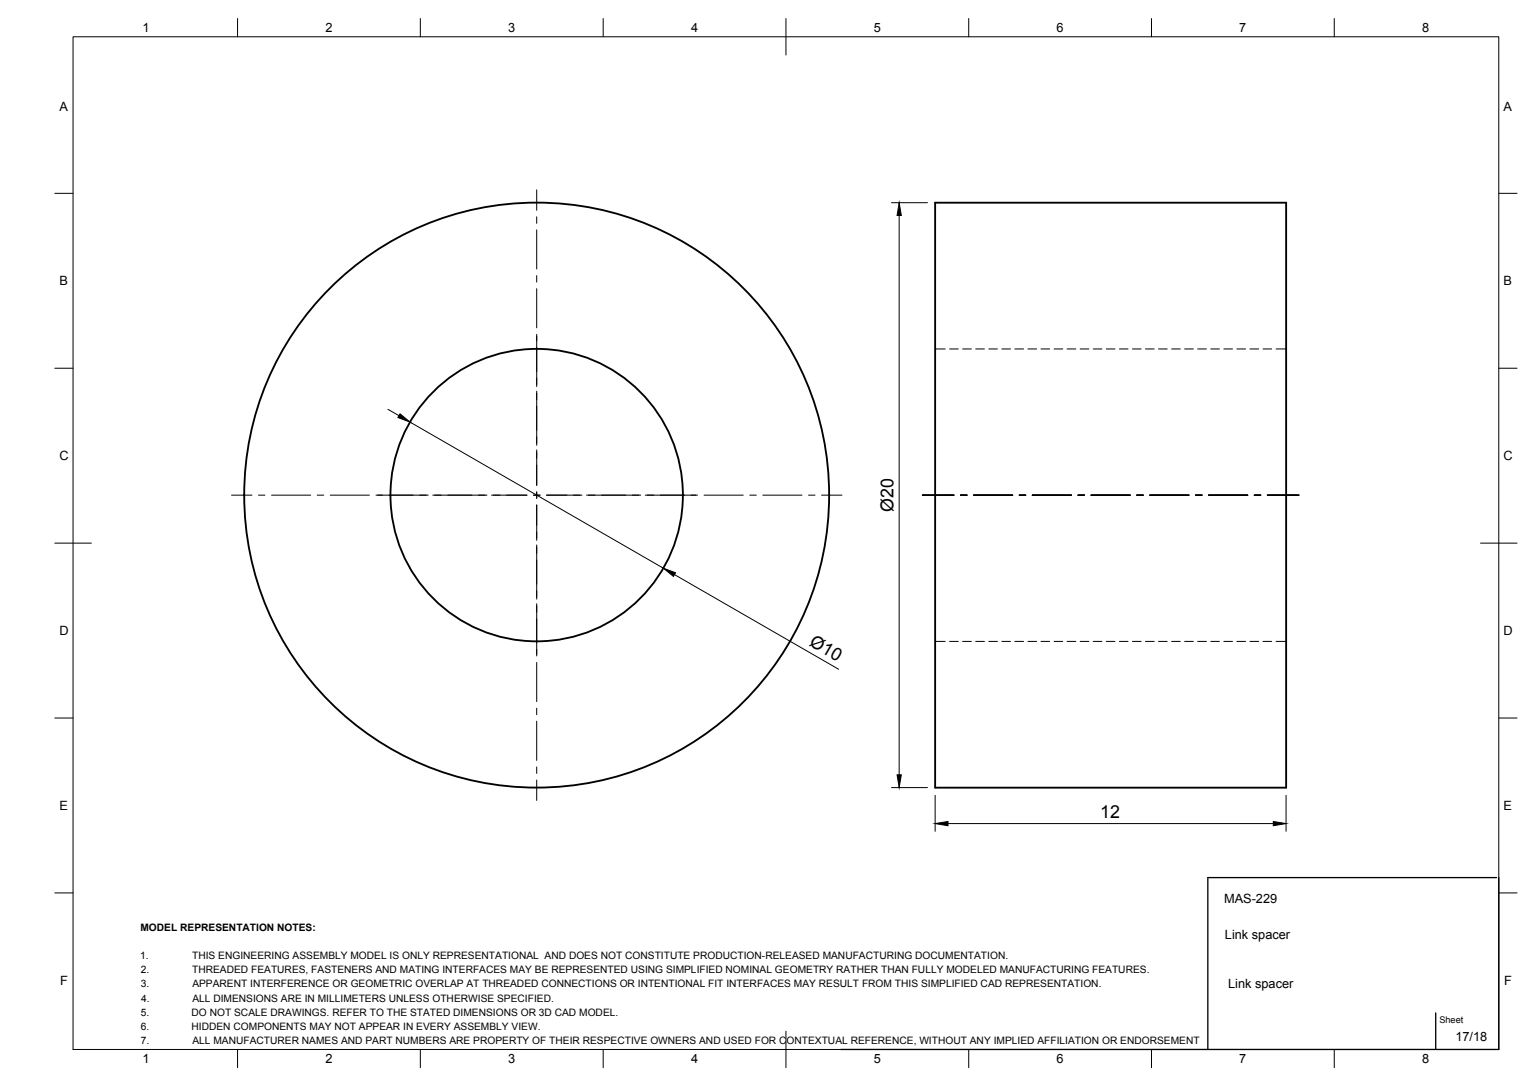
ISO-10303-21;
HEADER;
/* Generated by software containing ST-Developer
 * from STEP Tools, Inc. (www.steptools.com) 
 */

FILE_DESCRIPTION(
/* description */ ('Independently dimensioned six-bar single-leg walking-linkage demonstr
ator. Whole-mm20 crank,60 upper rocker,80/120 ternary coupler,120 lowe
r rocker,140 knee pitch and260 toe reach; ground pivots0/0,60/0,40/60.
 Seven native revolutes close both loops. Four reused native library f
amilies, fully retained shared pins and layered real spacer stacks, bo
nded rubber toe. Benchtop reference mechanism; no complete vehicle, lo
ad, gait stability, adhesive, weld, fit or life rating.'),
/* implementation_level */ '2;1');

FILE_NAME(
/* name */ 'Link spacer.step',
/* time_stamp */ '2026-11-09T20:33:14-08:00',
/* author */ (''),
/* organization */ (''),
/* preprocessor_version */ 'ST-DEVELOPER v20.2',
/* originating_system */ 'Autodesk Translation Framework v15.17.0.0',
/* authorisation */ '');

FILE_SCHEMA (('AUTOMOTIVE_DESIGN { 1 0 10303 214 3 1 1 }'));
ENDSEC;

DATA;
#10=MECHANICAL_DESIGN_GEOMETRIC_PRESENTATION_REPRESENTATION('',(#272),#4048);
#236=SHAPE_REPRESENTATION_RELATIONSHIP('SRR','None',#4160,#254);
#254=ADVANCED_BREP_SHAPE_REPRESENTATION('',(#290),#4047);
#272=STYLED_ITEM('',(#4253),#290);
#290=MANIFOLD_SOLID_BREP('Body1',#2161);
#346=FACE_BOUND('',#721,.T.);
#347=FACE_BOUND('',#723,.T.);
#413=PLANE('',#2618);
#414=PLANE('',#2619);
#537=FACE_OUTER_BOUND('',#718,.T.);
#538=FACE_OUTER_BOUND('',#719,.T.);
#539=FACE_OUTER_BOUND('',#720,.T.);
#540=FACE_OUTER_BOUND('',#722,.T.);
#718=EDGE_LOOP('',(#1951,#1952,#1953,#1954));
#719=EDGE_LOOP('',(#1955,#1956,#1957,#1958));
#720=EDGE_LOOP('',(#1959));
#721=EDGE_LOOP('',(#1960));
#722=EDGE_LOOP('',(#1961));
#723=EDGE_LOOP('',(#1962));
#847=LINE('',#3948,#972);
#848=LINE('',#3954,#973);
#972=VECTOR('',#3300,5.);
#973=VECTOR('',#3307,10.);
#1084=CIRCLE('',#2613,5.);
#1085=CIRCLE('',#2614,5.);
#1086=CIRCLE('',#2616,10.);
#1087=CIRCLE('',#2617,10.);
#1242=VERTEX_POINT('',#3945);
#1243=VERTEX_POINT('',#3947);
#1244=VERTEX_POINT('',#3951);
#1245=VERTEX_POINT('',#3953);
#1479=EDGE_CURVE('',#1242,#1242,#1084,.T.);
#1480=EDGE_CURVE('',#1242,#1243,#847,.T.);
#1481=EDGE_CURVE('',#1243,#1243,#1085,.T.);
#1482=EDGE_CURVE('',#1244,#1244,#1086,.T.);
#1483=EDGE_CURVE('',#1244,#1245,#848,.T.);
#1484=EDGE_CURVE('',#1245,#1245,#1087,.T.);
#1951=ORIENTED_EDGE('',*,*,#1479,.F.);
#1952=ORIENTED_EDGE('',*,*,#1480,.T.);
#1953=ORIENTED_EDGE('',*,*,#1481,.T.);
#1954=ORIENTED_EDGE('',*,*,#1480,.F.);
#1955=ORIENTED_EDGE('',*,*,#1482,.F.);
#1956=ORIENTED_EDGE('',*,*,#1483,.T.);
#1957=ORIENTED_EDGE('',*,*,#1484,.T.);
#1958=ORIENTED_EDGE('',*,*,#1483,.F.);
#1959=ORIENTED_EDGE('',*,*,#1482,.T.);
#1960=ORIENTED_EDGE('',*,*,#1479,.T.);
#1961=ORIENTED_EDGE('',*,*,#1484,.F.);
#1962=ORIENTED_EDGE('',*,*,#1481,.F.);
#2016=CYLINDRICAL_SURFACE('',#2612,5.);
#2017=CYLINDRICAL_SURFACE('',#2615,10.);
#2140=ADVANCED_FACE('',(#537),#2016,.F.);
#2141=ADVANCED_FACE('',(#538),#2017,.T.);
#2142=ADVANCED_FACE('',(#539,#346),#413,.T.);
#2143=ADVANCED_FACE('',(#540,#347),#414,.F.);
#2161=CLOSED_SHELL('',(#2140,#2141,#2142,#2143));
#2611=AXIS2_PLACEMENT_3D('',#3943,#3294,#3295);
#2612=AXIS2_PLACEMENT_3D('',#3944,#3296,#3297);
#2613=AXIS2_PLACEMENT_3D('',#3946,#3298,#3299);
#2614=AXIS2_PLACEMENT_3D('',#3949,#3301,#3302);
#2615=AXIS2_PLACEMENT_3D('',#3950,#3303,#3304);
#2616=AXIS2_PLACEMENT_3D('',#3952,#3305,#3306);
#2617=AXIS2_PLACEMENT_3D('',#3955,#3308,#3309);
#2618=AXIS2_PLACEMENT_3D('',#3956,#3310,#3311);
#2619=AXIS2_PLACEMENT_3D('',#3957,#3312,#3313);
#3294=DIRECTION('axis',(0.,0.,1.));
#3295=DIRECTION('refdir',(1.,0.,0.));
#3296=DIRECTION('center_axis',(0.,0.,1.));
#3297=DIRECTION('ref_axis',(1.,0.,0.));
#3298=DIRECTION('center_axis',(0.,0.,-1.));
#3299=DIRECTION('ref_axis',(1.,0.,0.));
#3300=DIRECTION('',(0.,0.,-1.));
#3301=DIRECTION('center_axis',(0.,0.,-1.));
#3302=DIRECTION('ref_axis',(1.,0.,0.));
#3303=DIRECTION('center_axis',(0.,0.,1.));
#3304=DIRECTION('ref_axis',(1.,0.,0.));
#3305=DIRECTION('center_axis',(0.,0.,1.));
#3306=DIRECTION('ref_axis',(1.,0.,0.));
#3307=DIRECTION('',(0.,0.,-1.));
#3308=DIRECTION('center_axis',(0.,0.,1.));
#3309=DIRECTION('ref_axis',(1.,0.,0.));
#3310=DIRECTION('center_axis',(0.,0.,1.));
#3311=DIRECTION('ref_axis',(1.,0.,0.));
#3312=DIRECTION('center_axis',(0.,0.,1.));
#3313=DIRECTION('ref_axis',(1.,0.,0.));
#3943=CARTESIAN_POINT('',(0.,0.,0.));
#3944=CARTESIAN_POINT('Origin',(0.,0.,0.));
#3945=CARTESIAN_POINT('',(-5.,-6.12323399573677E-16,12.));
#3946=CARTESIAN_POINT('Origin',(0.,0.,12.));
#3947=CARTESIAN_POINT('',(-5.,-6.12323399573677E-16,0.));
#3948=CARTESIAN_POINT('',(-5.,-6.12323399573677E-16,0.));
#3949=CARTESIAN_POINT('Origin',(0.,0.,0.));
#3950=CARTESIAN_POINT('Origin',(0.,0.,0.));
#3951=CARTESIAN_POINT('',(-10.,-1.22464679914735E-15,12.));
#3952=CARTESIAN_POINT('Origin',(0.,0.,12.));
#3953=CARTESIAN_POINT('',(-10.,-1.22464679914735E-15,0.));
#3954=CARTESIAN_POINT('',(-10.,-1.22464679914735E-15,0.));
#3955=CARTESIAN_POINT('Origin',(0.,0.,0.));
#3956=CARTESIAN_POINT('Origin',(0.,0.,12.));
#3957=CARTESIAN_POINT('Origin',(0.,0.,0.));
#4027=UNCERTAINTY_MEASURE_WITH_UNIT(LENGTH_MEASURE(0.01),#4049,
'DISTANCE_ACCURACY_VALUE',
'Maximum model space distance between geometric entities at asserted c
onnectivities');
#4028=UNCERTAINTY_MEASURE_WITH_UNIT(LENGTH_MEASURE(0.01),#4049,
'DISTANCE_ACCURACY_VALUE',
'Maximum model space distance between geometric entities at asserted c
onnectivities');
#4047=(
GEOMETRIC_REPRESENTATION_CONTEXT(3)
GLOBAL_UNCERTAINTY_ASSIGNED_CONTEXT((#4027))
GLOBAL_UNIT_ASSIGNED_CONTEXT((#4049,#4051,#4052))
REPRESENTATION_CONTEXT('','3D')
);
#4048=(
GEOMETRIC_REPRESENTATION_CONTEXT(3)
GLOBAL_UNCERTAINTY_ASSIGNED_CONTEXT((#4028))
GLOBAL_UNIT_ASSIGNED_CONTEXT((#4049,#4051,#4052))
REPRESENTATION_CONTEXT('','3D')
);
#4049=(
LENGTH_UNIT()
NAMED_UNIT(*)
SI_UNIT(.MILLI.,.METRE.)
);
#4051=(
NAMED_UNIT(*)
PLANE_ANGLE_UNIT()
SI_UNIT($,.RADIAN.)
);
#4052=(
NAMED_UNIT(*)
SI_UNIT($,.STERADIAN.)
SOLID_ANGLE_UNIT()
);
#4071=SHAPE_DEFINITION_REPRESENTATION(#4090,#4160);
#4090=PRODUCT_DEFINITION_SHAPE('',$,#4180);
#4160=SHAPE_REPRESENTATION('',(#2611),#4047);
#4161=PRODUCT_DEFINITION_CONTEXT('part definition',#4220,'design');
#4180=PRODUCT_DEFINITION('Link spacer','Link spacer',#4199,#4161);
#4199=PRODUCT_DEFINITION_FORMATION('',$,#4240);
#4220=APPLICATION_CONTEXT(
'Core Data for Automotive Mechanical Design Process');
#4221=PRODUCT_CONTEXT('part definition',#4220,'mechanical');
#4240=PRODUCT('Link spacer','Link spacer','Link spacer',(#4221));
#4253=PRESENTATION_STYLE_ASSIGNMENT((#4267));
#4267=SURFACE_STYLE_USAGE(.BOTH.,#4281);
#4281=SURFACE_SIDE_STYLE('',(#4295));
#4295=SURFACE_STYLE_FILL_AREA(#4309);
#4309=FILL_AREA_STYLE('Spacer gray',(#4323));
#4323=FILL_AREA_STYLE_COLOUR('Spacer gray',#4337);
#4337=COLOUR_RGB('Spacer gray',0.576470588235294,0.615686274509804,0.666666666666667);
ENDSEC;
END-ISO-10303-21;
